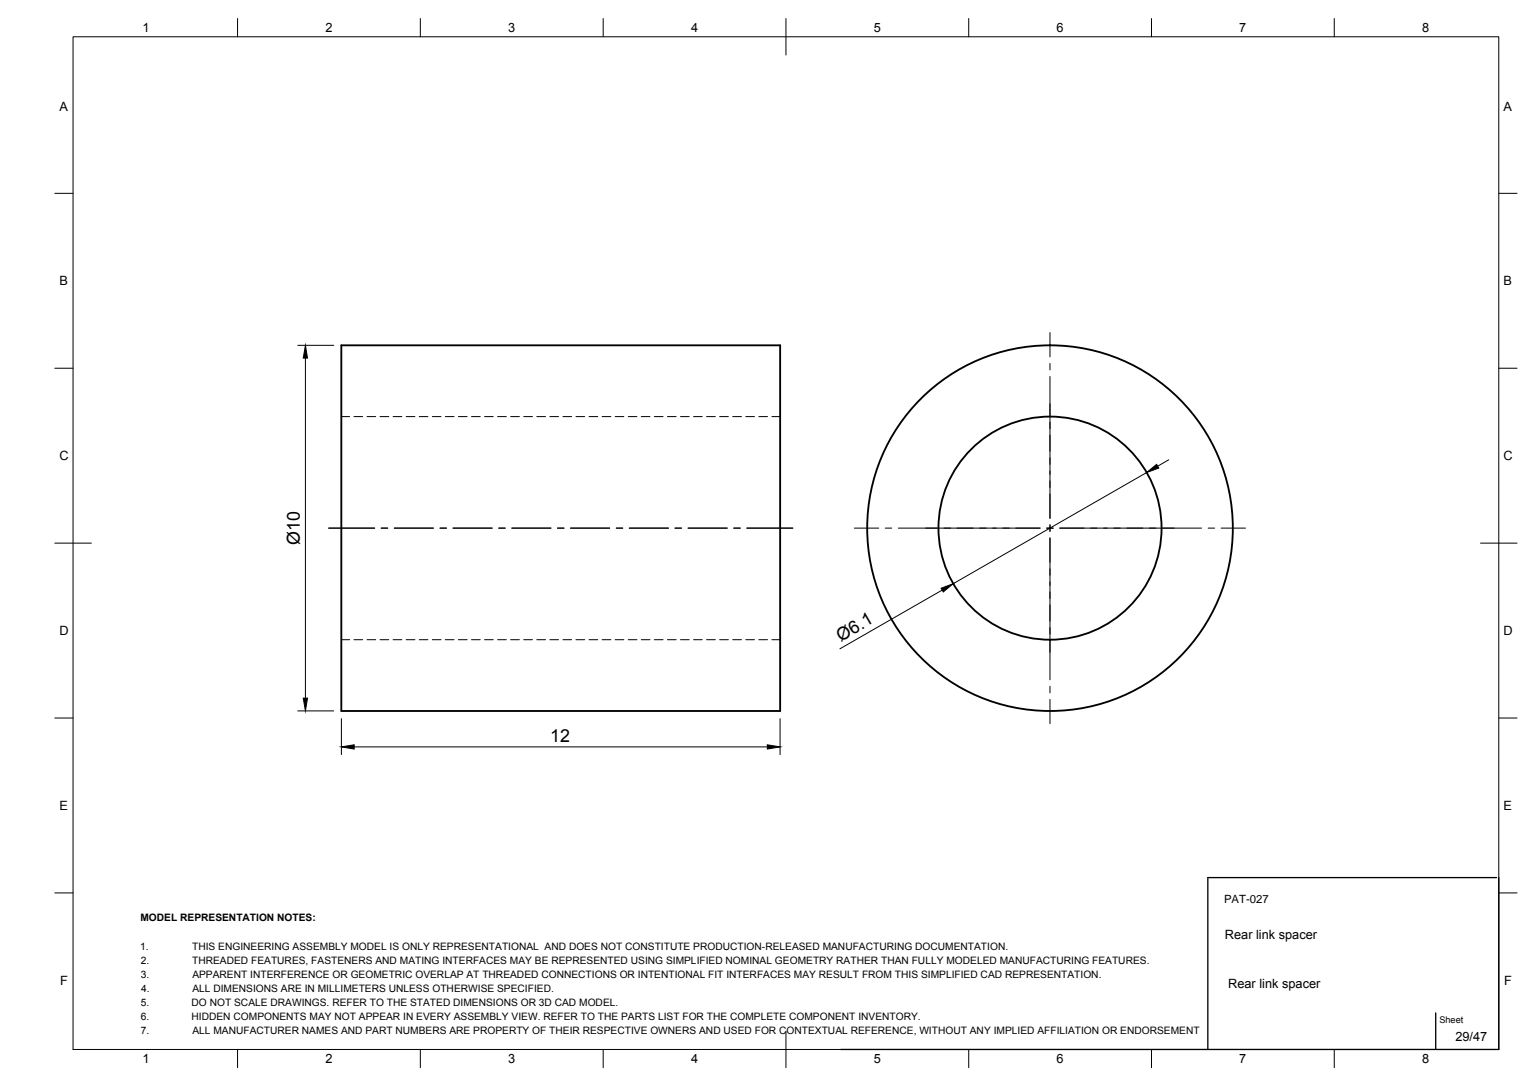
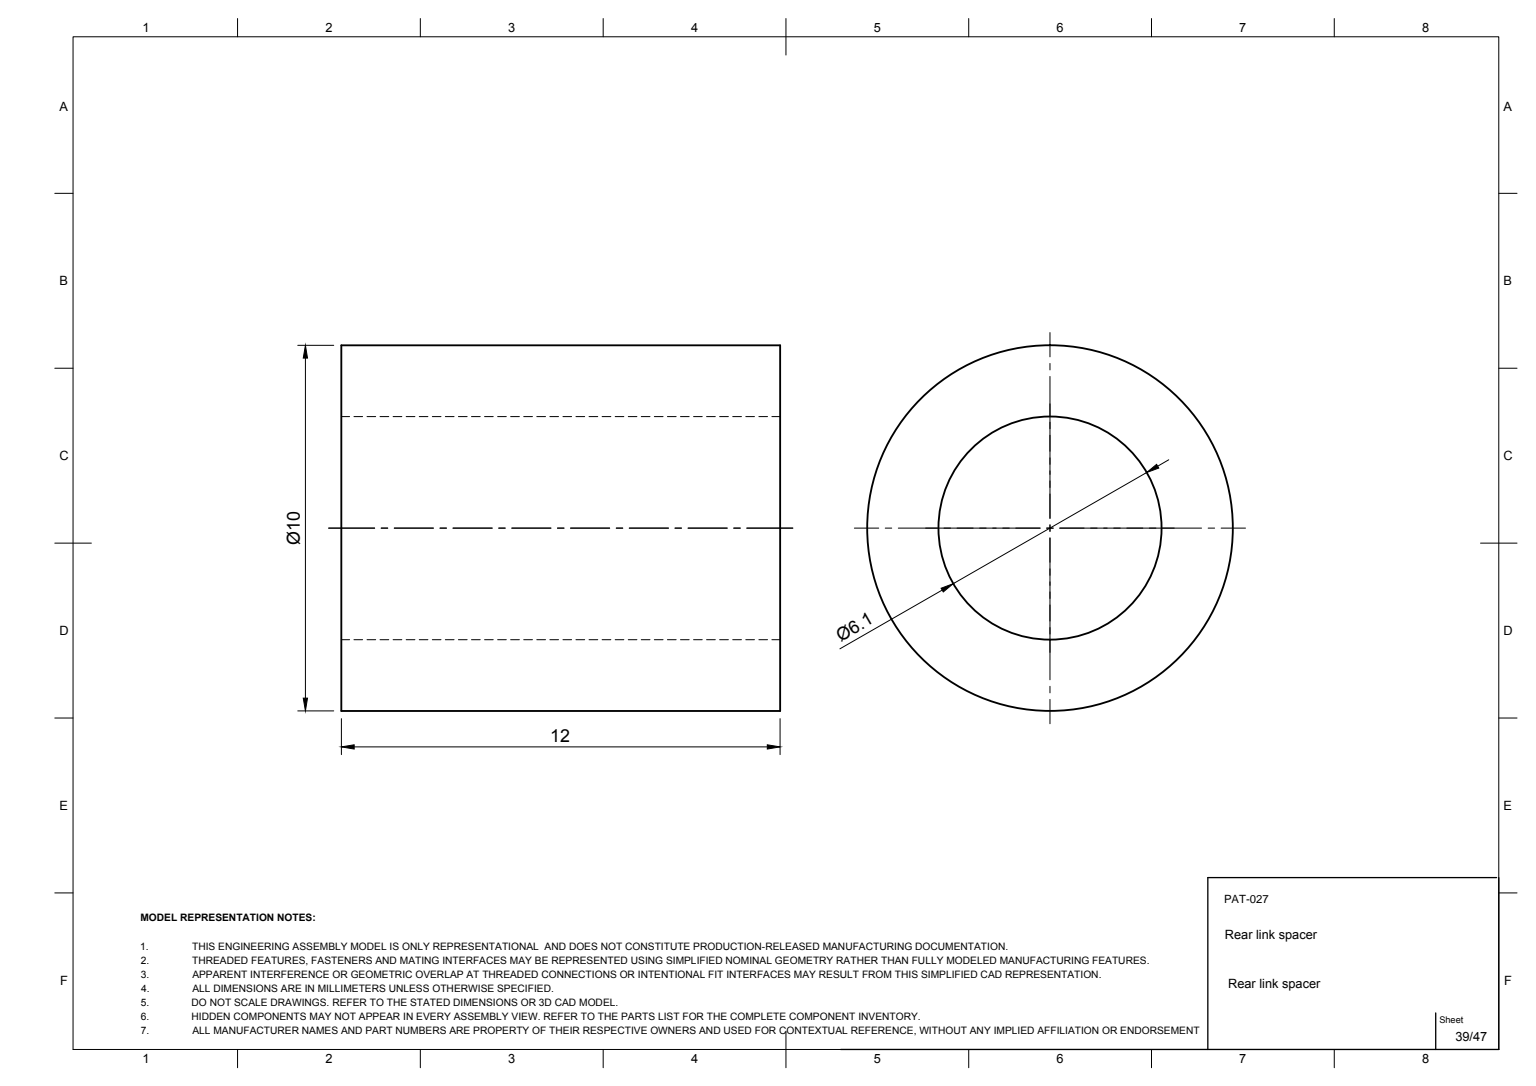
ISO-10303-21;
HEADER;
/* Generated by software containing ST-Developer
 * from STEP Tools, Inc. (www.steptools.com) 
 */

FILE_DESCRIPTION(
/* description */ ('Crank-driven oscillating fan base (mechanism only)'),

/* implementation_level */ '2;1');

FILE_NAME(
/* name */ 'Rear link spacer.step',
/* time_stamp */ '2026-10-28T03:25:00-07:00',
/* author */ (''),
/* organization */ (''),
/* preprocessor_version */ 'ST-DEVELOPER v20.2',
/* originating_system */ 'Autodesk Translation Framework v15.17.0.0',
/* authorisation */ '');

FILE_SCHEMA (('AUTOMOTIVE_DESIGN { 1 0 10303 214 3 1 1 }'));
ENDSEC;

DATA;
#10=MECHANICAL_DESIGN_GEOMETRIC_PRESENTATION_REPRESENTATION('',(#466),#11916);
#378=SHAPE_REPRESENTATION_RELATIONSHIP('SRR','None',#12104,#418);
#418=ADVANCED_BREP_SHAPE_REPRESENTATION('',(#513),#11895);
#466=STYLED_ITEM('',(#12389),#513);
#513=MANIFOLD_SOLID_BREP('Body1',#6097);
#640=FACE_BOUND('',#1601,.T.);
#641=FACE_BOUND('',#1603,.T.);
#798=PLANE('',#7078);
#799=PLANE('',#7079);
#1113=FACE_OUTER_BOUND('',#1598,.T.);
#1114=FACE_OUTER_BOUND('',#1599,.T.);
#1115=FACE_OUTER_BOUND('',#1600,.T.);
#1116=FACE_OUTER_BOUND('',#1602,.T.);
#1598=EDGE_LOOP('',(#5000,#5001,#5002,#5003));
#1599=EDGE_LOOP('',(#5004,#5005,#5006,#5007));
#1600=EDGE_LOOP('',(#5008));
#1601=EDGE_LOOP('',(#5009));
#1602=EDGE_LOOP('',(#5010));
#1603=EDGE_LOOP('',(#5011));
#1973=LINE('',#11085,#2306);
#1974=LINE('',#11091,#2307);
#2306=VECTOR('',#8616,0.305);
#2307=VECTOR('',#8623,0.5);
#2719=CIRCLE('',#7073,0.305);
#2720=CIRCLE('',#7074,0.305);
#2721=CIRCLE('',#7076,0.5);
#2722=CIRCLE('',#7077,0.5);
#3150=VERTEX_POINT('',#11082);
#3151=VERTEX_POINT('',#11084);
#3152=VERTEX_POINT('',#11088);
#3153=VERTEX_POINT('',#11090);
#3795=EDGE_CURVE('',#3150,#3150,#2719,.T.);
#3796=EDGE_CURVE('',#3150,#3151,#1973,.T.);
#3797=EDGE_CURVE('',#3151,#3151,#2720,.T.);
#3798=EDGE_CURVE('',#3152,#3152,#2721,.T.);
#3799=EDGE_CURVE('',#3152,#3153,#1974,.T.);
#3800=EDGE_CURVE('',#3153,#3153,#2722,.T.);
#5000=ORIENTED_EDGE('',*,*,#3795,.F.);
#5001=ORIENTED_EDGE('',*,*,#3796,.T.);
#5002=ORIENTED_EDGE('',*,*,#3797,.T.);
#5003=ORIENTED_EDGE('',*,*,#3796,.F.);
#5004=ORIENTED_EDGE('',*,*,#3798,.F.);
#5005=ORIENTED_EDGE('',*,*,#3799,.T.);
#5006=ORIENTED_EDGE('',*,*,#3800,.T.);
#5007=ORIENTED_EDGE('',*,*,#3799,.F.);
#5008=ORIENTED_EDGE('',*,*,#3798,.T.);
#5009=ORIENTED_EDGE('',*,*,#3795,.T.);
#5010=ORIENTED_EDGE('',*,*,#3800,.F.);
#5011=ORIENTED_EDGE('',*,*,#3797,.F.);
#5642=CYLINDRICAL_SURFACE('',#7072,0.305);
#5643=CYLINDRICAL_SURFACE('',#7075,0.5);
#5919=ADVANCED_FACE('',(#1113),#5642,.F.);
#5920=ADVANCED_FACE('',(#1114),#5643,.T.);
#5921=ADVANCED_FACE('',(#1115,#640),#798,.T.);
#5922=ADVANCED_FACE('',(#1116,#641),#799,.F.);
#6097=CLOSED_SHELL('',(#5919,#5920,#5921,#5922));
#7071=AXIS2_PLACEMENT_3D('',#11080,#8610,#8611);
#7072=AXIS2_PLACEMENT_3D('',#11081,#8612,#8613);
#7073=AXIS2_PLACEMENT_3D('',#11083,#8614,#8615);
#7074=AXIS2_PLACEMENT_3D('',#11086,#8617,#8618);
#7075=AXIS2_PLACEMENT_3D('',#11087,#8619,#8620);
#7076=AXIS2_PLACEMENT_3D('',#11089,#8621,#8622);
#7077=AXIS2_PLACEMENT_3D('',#11092,#8624,#8625);
#7078=AXIS2_PLACEMENT_3D('',#11093,#8626,#8627);
#7079=AXIS2_PLACEMENT_3D('',#11094,#8628,#8629);
#8610=DIRECTION('axis',(0.,0.,1.));
#8611=DIRECTION('refdir',(1.,0.,0.));
#8612=DIRECTION('center_axis',(0.,0.,1.));
#8613=DIRECTION('ref_axis',(1.,0.,0.));
#8614=DIRECTION('center_axis',(0.,0.,-1.));
#8615=DIRECTION('ref_axis',(1.,0.,0.));
#8616=DIRECTION('',(0.,0.,-1.));
#8617=DIRECTION('center_axis',(0.,0.,-1.));
#8618=DIRECTION('ref_axis',(1.,0.,0.));
#8619=DIRECTION('center_axis',(0.,0.,1.));
#8620=DIRECTION('ref_axis',(1.,0.,0.));
#8621=DIRECTION('center_axis',(0.,0.,1.));
#8622=DIRECTION('ref_axis',(1.,0.,0.));
#8623=DIRECTION('',(0.,0.,-1.));
#8624=DIRECTION('center_axis',(0.,0.,1.));
#8625=DIRECTION('ref_axis',(1.,0.,0.));
#8626=DIRECTION('center_axis',(0.,0.,1.));
#8627=DIRECTION('ref_axis',(1.,0.,0.));
#8628=DIRECTION('center_axis',(0.,0.,1.));
#8629=DIRECTION('ref_axis',(1.,0.,0.));
#11080=CARTESIAN_POINT('',(0.,0.,0.));
#11081=CARTESIAN_POINT('Origin',(-0.429855350392604,2.61349944954989,7.4));
#11082=CARTESIAN_POINT('',(-0.734855350392604,2.61349944954989,8.6));
#11083=CARTESIAN_POINT('Origin',(-0.429855350392604,2.61349944954989,8.6));
#11084=CARTESIAN_POINT('',(-0.734855350392604,2.61349944954989,7.4));
#11085=CARTESIAN_POINT('',(-0.734855350392604,2.61349944954989,7.4));
#11086=CARTESIAN_POINT('Origin',(-0.429855350392604,2.61349944954989,7.4));
#11087=CARTESIAN_POINT('Origin',(-0.429855350392604,2.61349944954989,7.4));
#11088=CARTESIAN_POINT('',(-0.929855350392604,2.61349944954989,8.6));
#11089=CARTESIAN_POINT('Origin',(-0.429855350392604,2.61349944954989,8.6));
#11090=CARTESIAN_POINT('',(-0.929855350392604,2.61349944954989,7.4));
#11091=CARTESIAN_POINT('',(-0.929855350392604,2.61349944954989,7.4));
#11092=CARTESIAN_POINT('Origin',(-0.429855350392604,2.61349944954989,7.4));
#11093=CARTESIAN_POINT('Origin',(-0.429855350392604,2.61349944954989,8.6));
#11094=CARTESIAN_POINT('Origin',(-0.429855350392604,2.61349944954989,7.4));
#11848=UNCERTAINTY_MEASURE_WITH_UNIT(LENGTH_MEASURE(0.001),#11917,
'DISTANCE_ACCURACY_VALUE',
'Maximum model space distance between geometric entities at asserted c
onnectivities');
#11869=UNCERTAINTY_MEASURE_WITH_UNIT(LENGTH_MEASURE(0.001),#11917,
'DISTANCE_ACCURACY_VALUE',
'Maximum model space distance between geometric entities at asserted c
onnectivities');
#11895=(
GEOMETRIC_REPRESENTATION_CONTEXT(3)
GLOBAL_UNCERTAINTY_ASSIGNED_CONTEXT((#11848))
GLOBAL_UNIT_ASSIGNED_CONTEXT((#11917,#11919,#11920))
REPRESENTATION_CONTEXT('','3D')
);
#11916=(
GEOMETRIC_REPRESENTATION_CONTEXT(3)
GLOBAL_UNCERTAINTY_ASSIGNED_CONTEXT((#11869))
GLOBAL_UNIT_ASSIGNED_CONTEXT((#11917,#11919,#11920))
REPRESENTATION_CONTEXT('','3D')
);
#11917=(
LENGTH_UNIT()
NAMED_UNIT(*)
SI_UNIT(.CENTI.,.METRE.)
);
#11919=(
NAMED_UNIT(*)
PLANE_ANGLE_UNIT()
SI_UNIT($,.RADIAN.)
);
#11920=(
NAMED_UNIT(*)
SI_UNIT($,.STERADIAN.)
SOLID_ANGLE_UNIT()
);
#11946=SHAPE_DEFINITION_REPRESENTATION(#11997,#12104);
#11997=PRODUCT_DEFINITION_SHAPE('',$,#12151);
#12104=SHAPE_REPRESENTATION('',(#7071),#11895);
#12125=PRODUCT_DEFINITION_CONTEXT('part definition',#12265,'design');
#12151=PRODUCT_DEFINITION('Rear link spacer','Rear link spacer',#12197,
#12125);
#12197=PRODUCT_DEFINITION_FORMATION('',$,#12292);
#12265=APPLICATION_CONTEXT(
'Core Data for Automotive Mechanical Design Process');
#12266=PRODUCT_CONTEXT('part definition',#12265,'mechanical');
#12292=PRODUCT('Rear link spacer','Rear link spacer','Rear link spacer',
(#12266));
#12383=COLOUR_RGB('Off White',0.89,0.88,0.83);
#12384=FILL_AREA_STYLE_COLOUR('',#12383);
#12385=FILL_AREA_STYLE('',(#12384));
#12386=SURFACE_STYLE_FILL_AREA(#12385);
#12387=SURFACE_SIDE_STYLE('',(#12386));
#12388=SURFACE_STYLE_USAGE(.BOTH.,#12387);
#12389=PRESENTATION_STYLE_ASSIGNMENT((#12388));
ENDSEC;
END-ISO-10303-21;
